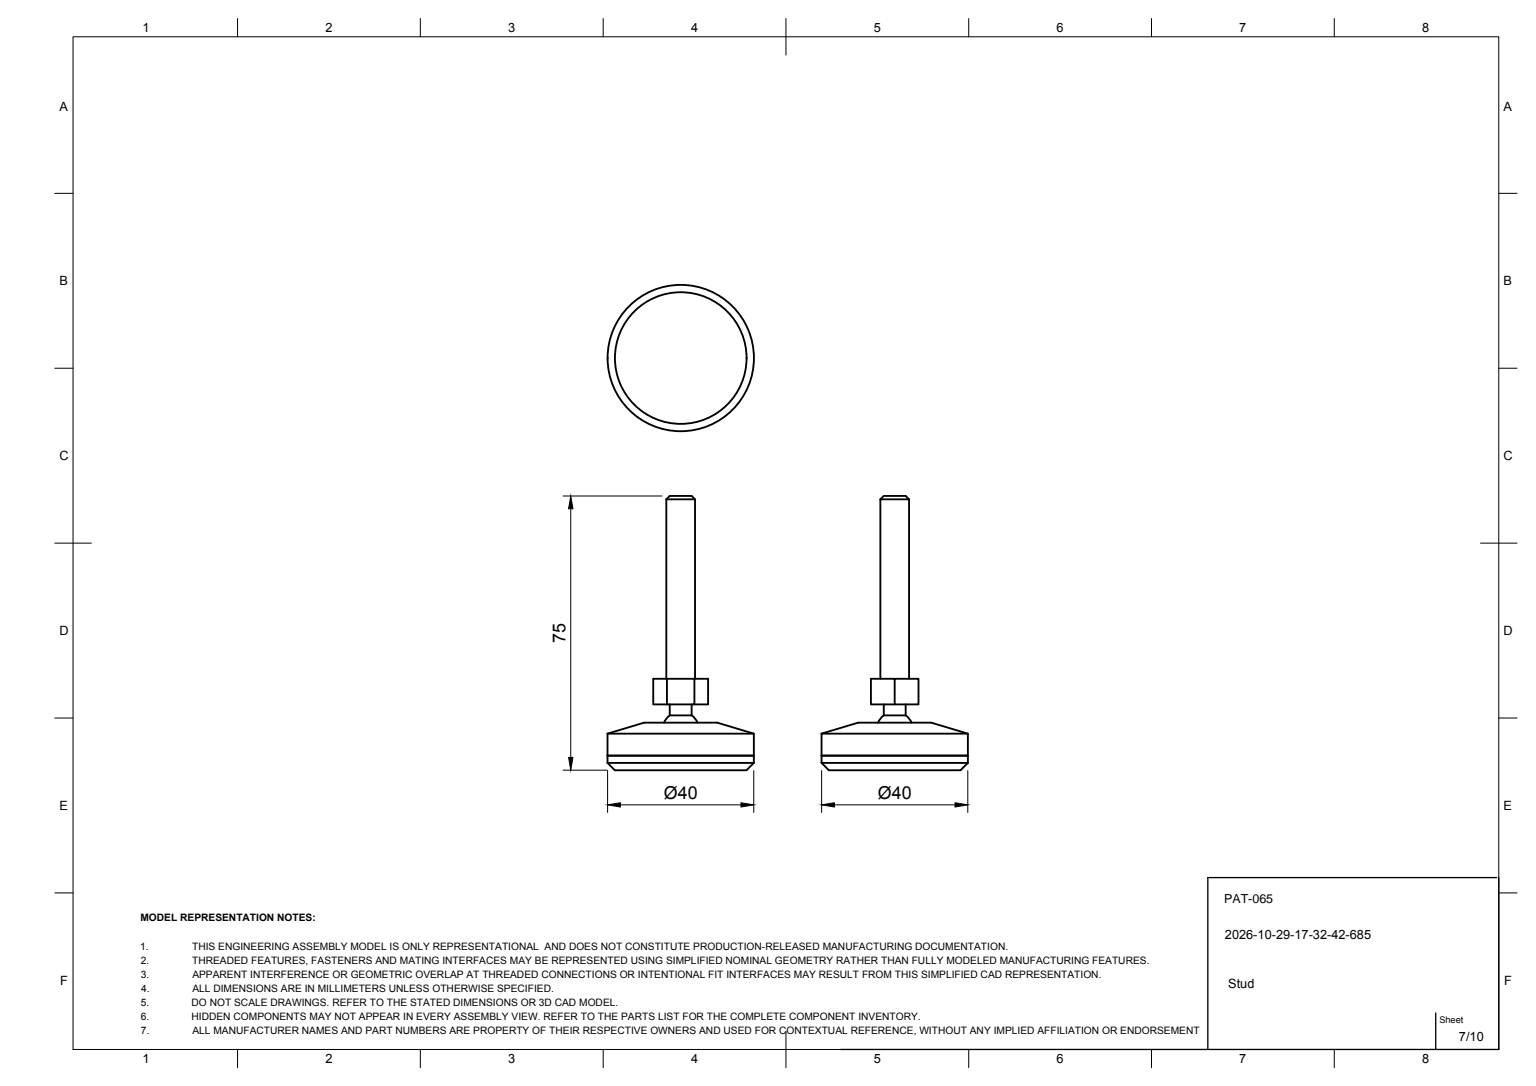
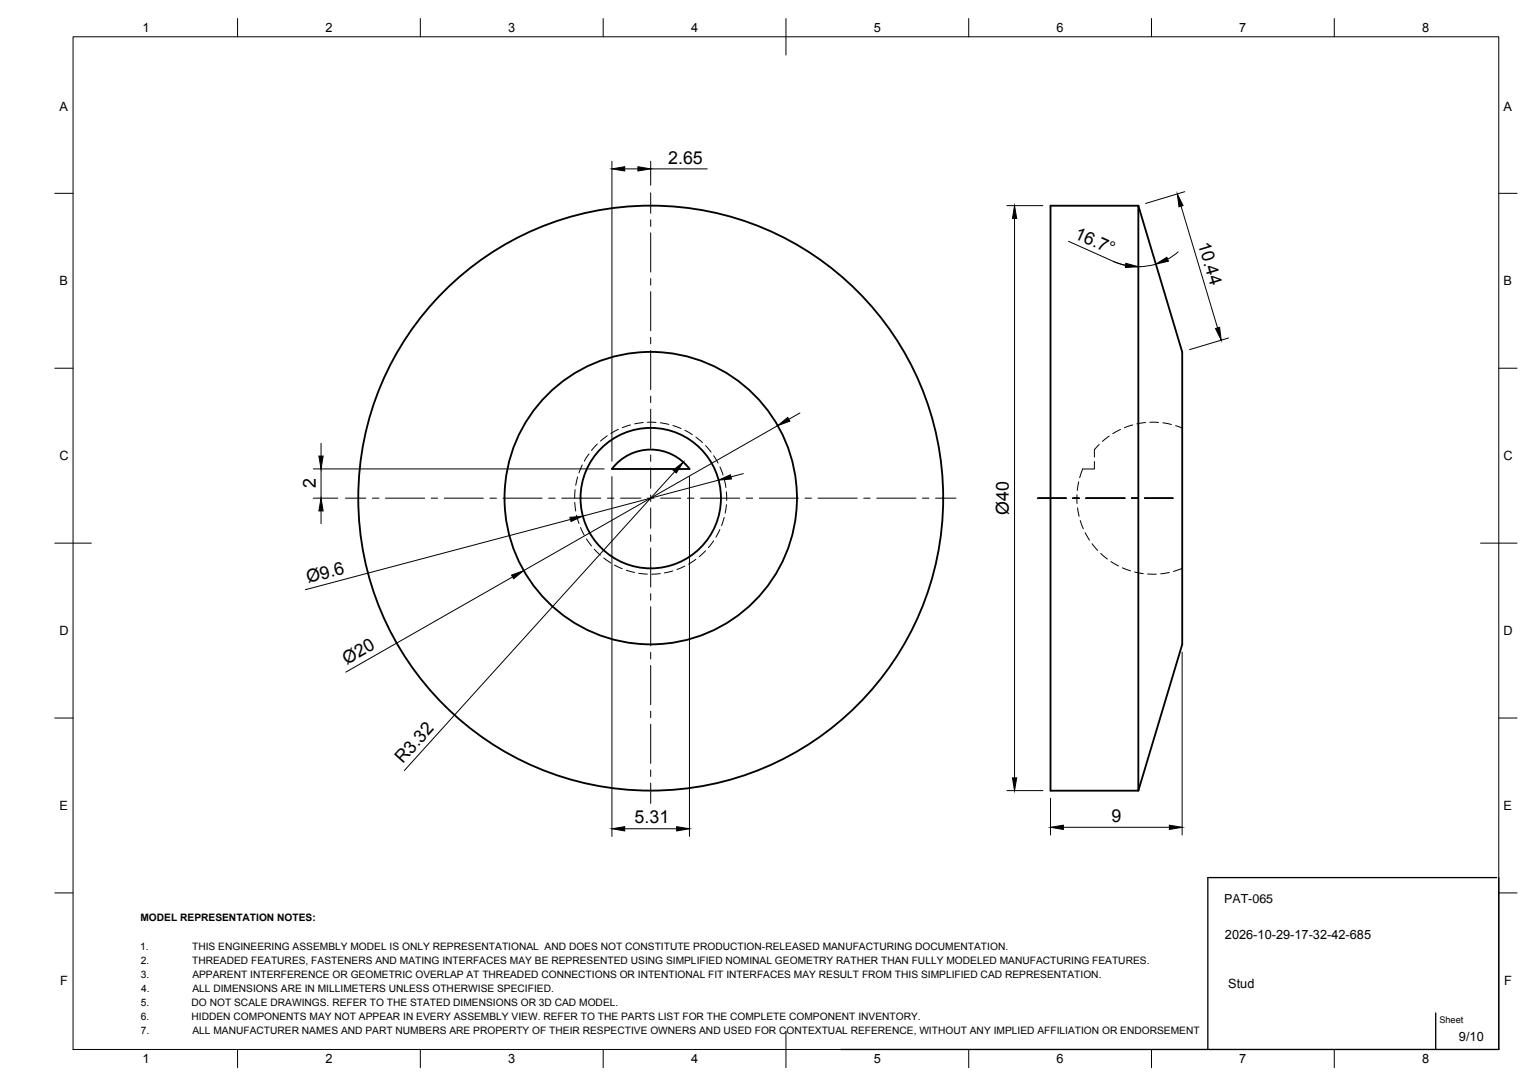
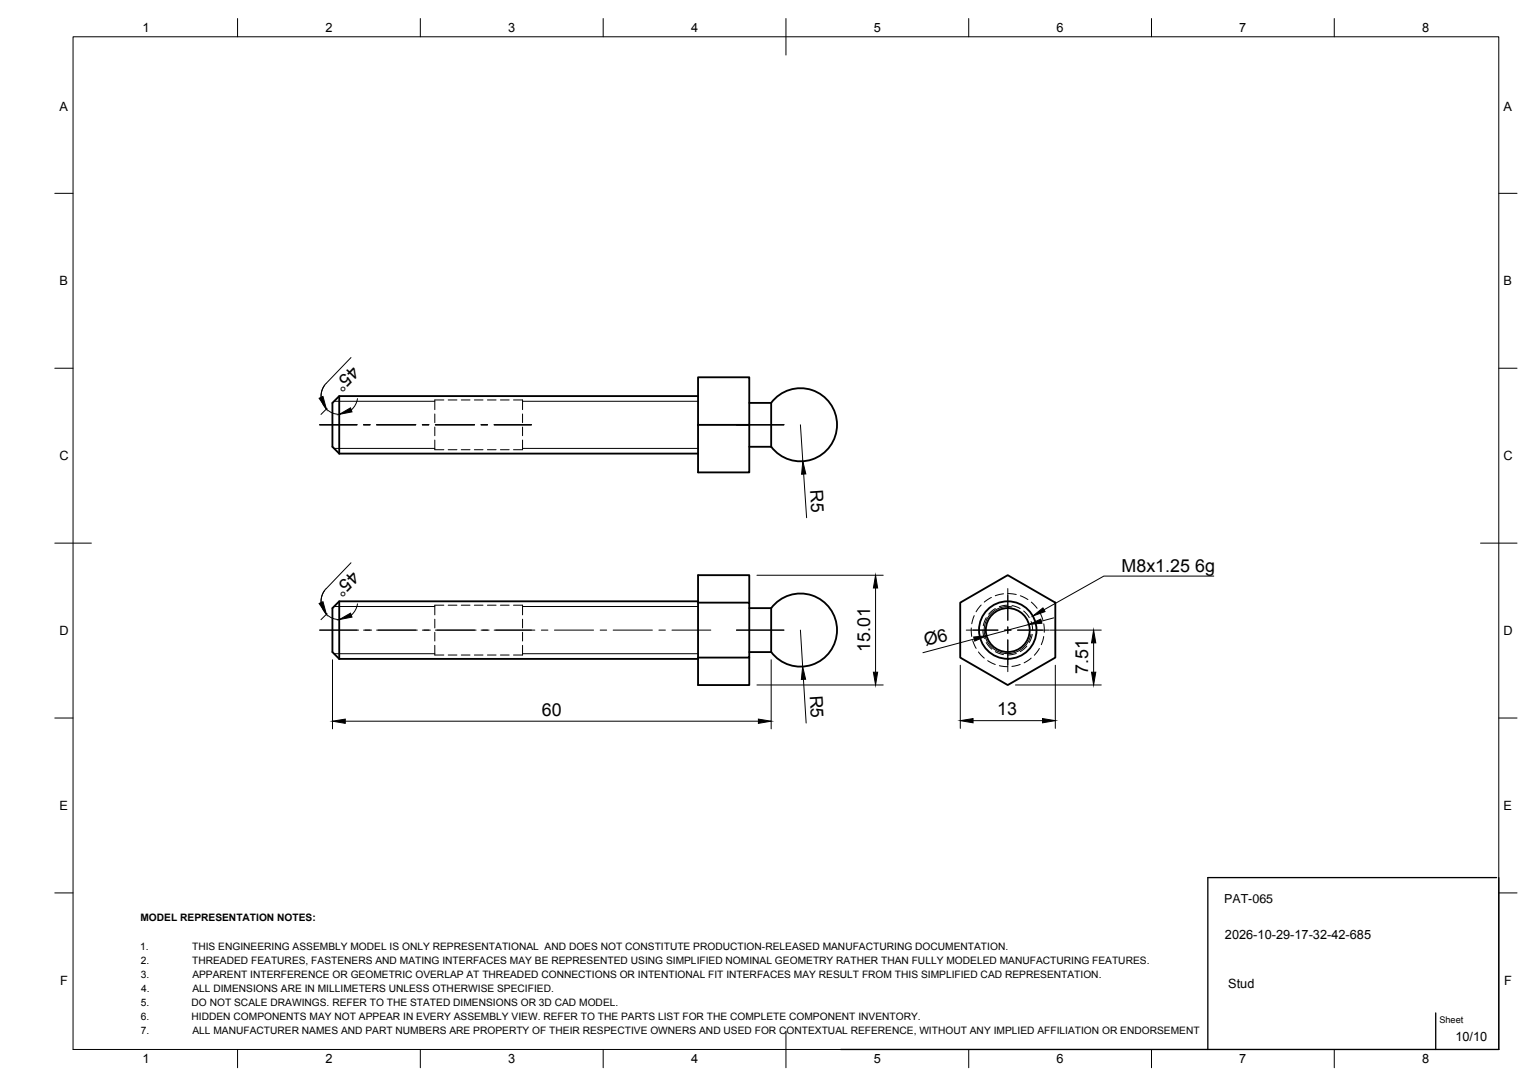
ISO-10303-21;
HEADER;
/* Generated by software containing ST-Developer
 * from STEP Tools, Inc. (www.steptools.com) 
 */

FILE_DESCRIPTION(
/* description */ ('PAT-065'),
/* implementation_level */ '2;1');

FILE_NAME(
/* name */ 'Stud.step',
/* time_stamp */ '2026-10-28T22:09:22-07:00',
/* author */ (''),
/* organization */ (''),
/* preprocessor_version */ 'ST-DEVELOPER v20.2',
/* originating_system */ 'Autodesk Translation Framework v15.17.0.0',
/* authorisation */ '');

FILE_SCHEMA (('AUTOMOTIVE_DESIGN { 1 0 10303 214 3 1 1 }'));
ENDSEC;

DATA;
#10=MECHANICAL_DESIGN_GEOMETRIC_PRESENTATION_REPRESENTATION('',(#164),#5502);
#115=ORIENTED_CLOSED_SHELL('',*,#3212,.F.);
#116=BREP_WITH_VOIDS('Body1',#3211,(#115));
#118=SPHERICAL_SURFACE('',#3514,0.5);
#123=CONICAL_SURFACE('',#3511,0.35,0.78539816339745);
#144=SHAPE_REPRESENTATION_RELATIONSHIP('SRR','None',#5562,#154);
#154=ADVANCED_BREP_SHAPE_REPRESENTATION('',(#116),#5498);
#164=STYLED_ITEM('',(#5701),#116);
#193=FACE_BOUND('',#641,.T.);
#194=FACE_BOUND('',#650,.T.);
#293=PLANE('',#3497);
#294=PLANE('',#3499);
#295=PLANE('',#3500);
#296=PLANE('',#3501);
#297=PLANE('',#3502);
#298=PLANE('',#3503);
#299=PLANE('',#3504);
#300=PLANE('',#3508);
#301=PLANE('',#3513);
#302=PLANE('',#3519);
#303=PLANE('',#3520);
#450=FACE_OUTER_BOUND('',#640,.T.);
#451=FACE_OUTER_BOUND('',#642,.T.);
#452=FACE_OUTER_BOUND('',#643,.T.);
#453=FACE_OUTER_BOUND('',#644,.T.);
#454=FACE_OUTER_BOUND('',#645,.T.);
#455=FACE_OUTER_BOUND('',#646,.T.);
#456=FACE_OUTER_BOUND('',#647,.T.);
#457=FACE_OUTER_BOUND('',#648,.T.);
#458=FACE_OUTER_BOUND('',#649,.T.);
#459=FACE_OUTER_BOUND('',#651,.T.);
#460=FACE_OUTER_BOUND('',#652,.T.);
#461=FACE_OUTER_BOUND('',#653,.T.);
#462=FACE_OUTER_BOUND('',#654,.T.);
#463=FACE_OUTER_BOUND('',#655,.T.);
#464=FACE_OUTER_BOUND('',#656,.T.);
#465=FACE_OUTER_BOUND('',#657,.T.);
#640=EDGE_LOOP('',(#2742,#2743,#2744,#2745,#2746,#2747));
#641=EDGE_LOOP('',(#2748));
#642=EDGE_LOOP('',(#2749,#2750,#2751,#2752));
#643=EDGE_LOOP('',(#2753,#2754,#2755,#2756));
#644=EDGE_LOOP('',(#2757,#2758,#2759,#2760));
#645=EDGE_LOOP('',(#2761,#2762,#2763,#2764));
#646=EDGE_LOOP('',(#2765,#2766,#2767,#2768));
#647=EDGE_LOOP('',(#2769,#2770,#2771,#2772));
#648=EDGE_LOOP('',(#2773,#2774,#2775,#2776));
#649=EDGE_LOOP('',(#2777,#2778,#2779,#2780,#2781,#2782));
#650=EDGE_LOOP('',(#2783));
#651=EDGE_LOOP('',(#2784,#2785,#2786,#2787));
#652=EDGE_LOOP('',(#2788,#2789,#2790,#2791));
#653=EDGE_LOOP('',(#2792));
#654=EDGE_LOOP('',(#2793,#2794,#2795));
#655=EDGE_LOOP('',(#2796,#2797,#2798,#2799));
#656=EDGE_LOOP('',(#2800));
#657=EDGE_LOOP('',(#2801));
#955=LINE('',#5152,#1286);
#956=LINE('',#5154,#1287);
#957=LINE('',#5156,#1288);
#958=LINE('',#5158,#1289);
#959=LINE('',#5160,#1290);
#960=LINE('',#5161,#1291);
#961=LINE('',#5167,#1292);
#962=LINE('',#5168,#1293);
#963=LINE('',#5169,#1294);
#964=LINE('',#5172,#1295);
#965=LINE('',#5173,#1296);
#966=LINE('',#5176,#1297);
#967=LINE('',#5177,#1298);
#968=LINE('',#5180,#1299);
#969=LINE('',#5181,#1300);
#970=LINE('',#5184,#1301);
#971=LINE('',#5185,#1302);
#972=LINE('',#5187,#1303);
#973=LINE('',#5192,#1304);
#974=LINE('',#5198,#1305);
#975=LINE('',#5202,#1306);
#976=LINE('',#5211,#1307);
#1286=VECTOR('',#4206,1.);
#1287=VECTOR('',#4207,1.);
#1288=VECTOR('',#4208,1.);
#1289=VECTOR('',#4209,1.);
#1290=VECTOR('',#4210,1.);
#1291=VECTOR('',#4211,1.);
#1292=VECTOR('',#4216,1.);
#1293=VECTOR('',#4217,1.);
#1294=VECTOR('',#4218,1.);
#1295=VECTOR('',#4221,1.);
#1296=VECTOR('',#4222,1.);
#1297=VECTOR('',#4225,1.);
#1298=VECTOR('',#4226,1.);
#1299=VECTOR('',#4229,1.);
#1300=VECTOR('',#4230,1.);
#1301=VECTOR('',#4233,1.);
#1302=VECTOR('',#4234,1.);
#1303=VECTOR('',#4237,1.);
#1304=VECTOR('',#4242,0.3);
#1305=VECTOR('',#4251,0.4);
#1306=VECTOR('',#4256,0.35);
#1307=VECTOR('',#4267,0.34);
#1415=CIRCLE('',#3498,0.3933);
#1416=CIRCLE('',#3506,0.3);
#1417=CIRCLE('',#3507,0.3);
#1418=CIRCLE('',#3510,0.3933);
#1419=CIRCLE('',#3512,0.3);
#1420=CIRCLE('',#3515,0.5);
#1421=CIRCLE('',#3517,0.34);
#1422=CIRCLE('',#3518,0.34);
#1640=VERTEX_POINT('',#5150);
#1641=VERTEX_POINT('',#5151);
#1642=VERTEX_POINT('',#5153);
#1643=VERTEX_POINT('',#5155);
#1644=VERTEX_POINT('',#5157);
#1645=VERTEX_POINT('',#5159);
#1646=VERTEX_POINT('',#5162);
#1647=VERTEX_POINT('',#5165);
#1648=VERTEX_POINT('',#5166);
#1649=VERTEX_POINT('',#5171);
#1650=VERTEX_POINT('',#5175);
#1651=VERTEX_POINT('',#5179);
#1652=VERTEX_POINT('',#5183);
#1653=VERTEX_POINT('',#5189);
#1654=VERTEX_POINT('',#5191);
#1655=VERTEX_POINT('',#5196);
#1656=VERTEX_POINT('',#5200);
#1657=VERTEX_POINT('',#5205);
#1658=VERTEX_POINT('',#5208);
#1659=VERTEX_POINT('',#5210);
#2021=EDGE_CURVE('',#1640,#1641,#955,.T.);
#2022=EDGE_CURVE('',#1641,#1642,#956,.T.);
#2023=EDGE_CURVE('',#1642,#1643,#957,.T.);
#2024=EDGE_CURVE('',#1643,#1644,#958,.T.);
#2025=EDGE_CURVE('',#1644,#1645,#959,.T.);
#2026=EDGE_CURVE('',#1645,#1640,#960,.T.);
#2027=EDGE_CURVE('',#1646,#1646,#1415,.F.);
#2028=EDGE_CURVE('',#1647,#1648,#961,.T.);
#2029=EDGE_CURVE('',#1648,#1640,#962,.T.);
#2030=EDGE_CURVE('',#1647,#1645,#963,.T.);
#2031=EDGE_CURVE('',#1649,#1647,#964,.T.);
#2032=EDGE_CURVE('',#1649,#1644,#965,.T.);
#2033=EDGE_CURVE('',#1650,#1649,#966,.T.);
#2034=EDGE_CURVE('',#1650,#1643,#967,.T.);
#2035=EDGE_CURVE('',#1651,#1650,#968,.T.);
#2036=EDGE_CURVE('',#1651,#1642,#969,.T.);
#2037=EDGE_CURVE('',#1652,#1651,#970,.T.);
#2038=EDGE_CURVE('',#1652,#1641,#971,.T.);
#2039=EDGE_CURVE('',#1648,#1652,#972,.T.);
#2040=EDGE_CURVE('',#1653,#1653,#1416,.T.);
#2041=EDGE_CURVE('',#1653,#1654,#973,.T.);
#2042=EDGE_CURVE('',#1654,#1654,#1417,.T.);
#2043=EDGE_CURVE('',#1655,#1655,#1418,.F.);
#2044=EDGE_CURVE('',#1655,#1646,#974,.T.);
#2045=EDGE_CURVE('',#1656,#1656,#1419,.T.);
#2046=EDGE_CURVE('',#1656,#1655,#975,.T.);
#2047=EDGE_CURVE('',#1654,#1657,#1420,.T.);
#2048=EDGE_CURVE('',#1658,#1658,#1421,.T.);
#2049=EDGE_CURVE('',#1658,#1659,#976,.T.);
#2050=EDGE_CURVE('',#1659,#1659,#1422,.T.);
#2742=ORIENTED_EDGE('',*,*,#2021,.T.);
#2743=ORIENTED_EDGE('',*,*,#2022,.T.);
#2744=ORIENTED_EDGE('',*,*,#2023,.T.);
#2745=ORIENTED_EDGE('',*,*,#2024,.T.);
#2746=ORIENTED_EDGE('',*,*,#2025,.T.);
#2747=ORIENTED_EDGE('',*,*,#2026,.T.);
#2748=ORIENTED_EDGE('',*,*,#2027,.F.);
#2749=ORIENTED_EDGE('',*,*,#2028,.T.);
#2750=ORIENTED_EDGE('',*,*,#2029,.T.);
#2751=ORIENTED_EDGE('',*,*,#2026,.F.);
#2752=ORIENTED_EDGE('',*,*,#2030,.F.);
#2753=ORIENTED_EDGE('',*,*,#2031,.T.);
#2754=ORIENTED_EDGE('',*,*,#2030,.T.);
#2755=ORIENTED_EDGE('',*,*,#2025,.F.);
#2756=ORIENTED_EDGE('',*,*,#2032,.F.);
#2757=ORIENTED_EDGE('',*,*,#2033,.T.);
#2758=ORIENTED_EDGE('',*,*,#2032,.T.);
#2759=ORIENTED_EDGE('',*,*,#2024,.F.);
#2760=ORIENTED_EDGE('',*,*,#2034,.F.);
#2761=ORIENTED_EDGE('',*,*,#2035,.T.);
#2762=ORIENTED_EDGE('',*,*,#2034,.T.);
#2763=ORIENTED_EDGE('',*,*,#2023,.F.);
#2764=ORIENTED_EDGE('',*,*,#2036,.F.);
#2765=ORIENTED_EDGE('',*,*,#2037,.T.);
#2766=ORIENTED_EDGE('',*,*,#2036,.T.);
#2767=ORIENTED_EDGE('',*,*,#2022,.F.);
#2768=ORIENTED_EDGE('',*,*,#2038,.F.);
#2769=ORIENTED_EDGE('',*,*,#2039,.T.);
#2770=ORIENTED_EDGE('',*,*,#2038,.T.);
#2771=ORIENTED_EDGE('',*,*,#2021,.F.);
#2772=ORIENTED_EDGE('',*,*,#2029,.F.);
#2773=ORIENTED_EDGE('',*,*,#2040,.F.);
#2774=ORIENTED_EDGE('',*,*,#2041,.T.);
#2775=ORIENTED_EDGE('',*,*,#2042,.F.);
#2776=ORIENTED_EDGE('',*,*,#2041,.F.);
#2777=ORIENTED_EDGE('',*,*,#2039,.F.);
#2778=ORIENTED_EDGE('',*,*,#2028,.F.);
#2779=ORIENTED_EDGE('',*,*,#2031,.F.);
#2780=ORIENTED_EDGE('',*,*,#2033,.F.);
#2781=ORIENTED_EDGE('',*,*,#2035,.F.);
#2782=ORIENTED_EDGE('',*,*,#2037,.F.);
#2783=ORIENTED_EDGE('',*,*,#2040,.T.);
#2784=ORIENTED_EDGE('',*,*,#2043,.F.);
#2785=ORIENTED_EDGE('',*,*,#2044,.T.);
#2786=ORIENTED_EDGE('',*,*,#2027,.T.);
#2787=ORIENTED_EDGE('',*,*,#2044,.F.);
#2788=ORIENTED_EDGE('',*,*,#2045,.F.);
#2789=ORIENTED_EDGE('',*,*,#2046,.T.);
#2790=ORIENTED_EDGE('',*,*,#2043,.T.);
#2791=ORIENTED_EDGE('',*,*,#2046,.F.);
#2792=ORIENTED_EDGE('',*,*,#2045,.T.);
#2793=ORIENTED_EDGE('',*,*,#2042,.T.);
#2794=ORIENTED_EDGE('',*,*,#2047,.T.);
#2795=ORIENTED_EDGE('',*,*,#2047,.F.);
#2796=ORIENTED_EDGE('',*,*,#2048,.F.);
#2797=ORIENTED_EDGE('',*,*,#2049,.T.);
#2798=ORIENTED_EDGE('',*,*,#2050,.T.);
#2799=ORIENTED_EDGE('',*,*,#2049,.F.);
#2800=ORIENTED_EDGE('',*,*,#2050,.F.);
#2801=ORIENTED_EDGE('',*,*,#2048,.T.);
#3020=CYLINDRICAL_SURFACE('',#3505,0.3);
#3021=CYLINDRICAL_SURFACE('',#3509,0.3933);
#3022=CYLINDRICAL_SURFACE('',#3516,0.34);
#3144=ADVANCED_FACE('',(#450,#193),#293,.T.);
#3145=ADVANCED_FACE('',(#451),#294,.T.);
#3146=ADVANCED_FACE('',(#452),#295,.T.);
#3147=ADVANCED_FACE('',(#453),#296,.T.);
#3148=ADVANCED_FACE('',(#454),#297,.T.);
#3149=ADVANCED_FACE('',(#455),#298,.T.);
#3150=ADVANCED_FACE('',(#456),#299,.T.);
#3151=ADVANCED_FACE('',(#457),#3020,.T.);
#3152=ADVANCED_FACE('',(#458,#194),#300,.T.);
#3153=ADVANCED_FACE('',(#459),#3021,.T.);
#3154=ADVANCED_FACE('',(#460),#123,.T.);
#3155=ADVANCED_FACE('',(#461),#301,.T.);
#3156=ADVANCED_FACE('',(#462),#118,.T.);
#3157=ADVANCED_FACE('',(#463),#3022,.F.);
#3158=ADVANCED_FACE('',(#464),#302,.F.);
#3159=ADVANCED_FACE('',(#465),#303,.T.);
#3211=CLOSED_SHELL('',(#3144,#3145,#3146,#3147,#3148,#3149,#3150,#3151,
#3152,#3153,#3154,#3155,#3156));
#3212=CLOSED_SHELL('',(#3157,#3158,#3159));
#3496=AXIS2_PLACEMENT_3D('',#5148,#4202,#4203);
#3497=AXIS2_PLACEMENT_3D('',#5149,#4204,#4205);
#3498=AXIS2_PLACEMENT_3D('',#5163,#4212,#4213);
#3499=AXIS2_PLACEMENT_3D('',#5164,#4214,#4215);
#3500=AXIS2_PLACEMENT_3D('',#5170,#4219,#4220);
#3501=AXIS2_PLACEMENT_3D('',#5174,#4223,#4224);
#3502=AXIS2_PLACEMENT_3D('',#5178,#4227,#4228);
#3503=AXIS2_PLACEMENT_3D('',#5182,#4231,#4232);
#3504=AXIS2_PLACEMENT_3D('',#5186,#4235,#4236);
#3505=AXIS2_PLACEMENT_3D('',#5188,#4238,#4239);
#3506=AXIS2_PLACEMENT_3D('',#5190,#4240,#4241);
#3507=AXIS2_PLACEMENT_3D('',#5193,#4243,#4244);
#3508=AXIS2_PLACEMENT_3D('',#5194,#4245,#4246);
#3509=AXIS2_PLACEMENT_3D('',#5195,#4247,#4248);
#3510=AXIS2_PLACEMENT_3D('',#5197,#4249,#4250);
#3511=AXIS2_PLACEMENT_3D('',#5199,#4252,#4253);
#3512=AXIS2_PLACEMENT_3D('',#5201,#4254,#4255);
#3513=AXIS2_PLACEMENT_3D('',#5203,#4257,#4258);
#3514=AXIS2_PLACEMENT_3D('',#5204,#4259,#4260);
#3515=AXIS2_PLACEMENT_3D('',#5206,#4261,#4262);
#3516=AXIS2_PLACEMENT_3D('',#5207,#4263,#4264);
#3517=AXIS2_PLACEMENT_3D('',#5209,#4265,#4266);
#3518=AXIS2_PLACEMENT_3D('',#5212,#4268,#4269);
#3519=AXIS2_PLACEMENT_3D('',#5213,#4270,#4271);
#3520=AXIS2_PLACEMENT_3D('',#5214,#4272,#4273);
#4202=DIRECTION('axis',(0.,0.,1.));
#4203=DIRECTION('refdir',(1.,0.,0.));
#4204=DIRECTION('center_axis',(0.,0.,1.));
#4205=DIRECTION('ref_axis',(1.,0.,0.));
#4206=DIRECTION('',(0.5,0.866025403784439,0.));
#4207=DIRECTION('',(-0.5,0.866025403784439,0.));
#4208=DIRECTION('',(-1.,1.4792020664489E-16,0.));
#4209=DIRECTION('',(-0.5,-0.866025403784439,0.));
#4210=DIRECTION('',(0.5,-0.866025403784439,0.));
#4211=DIRECTION('',(1.,-2.95840413289779E-16,0.));
#4212=DIRECTION('center_axis',(0.,0.,-1.));
#4213=DIRECTION('ref_axis',(1.,0.,0.));
#4214=DIRECTION('center_axis',(-2.95840413289779E-16,-1.,0.));
#4215=DIRECTION('ref_axis',(1.,-2.95840413289779E-16,0.));
#4216=DIRECTION('',(1.,-2.95840413289779E-16,0.));
#4217=DIRECTION('',(0.,0.,1.));
#4218=DIRECTION('',(0.,0.,1.));
#4219=DIRECTION('center_axis',(-0.866025403784439,-0.5,0.));
#4220=DIRECTION('ref_axis',(0.5,-0.866025403784439,0.));
#4221=DIRECTION('',(0.5,-0.866025403784439,0.));
#4222=DIRECTION('',(0.,0.,1.));
#4223=DIRECTION('center_axis',(-0.866025403784439,0.5,0.));
#4224=DIRECTION('ref_axis',(-0.5,-0.866025403784439,0.));
#4225=DIRECTION('',(-0.5,-0.866025403784439,0.));
#4226=DIRECTION('',(0.,0.,1.));
#4227=DIRECTION('center_axis',(1.4792020664489E-16,1.,0.));
#4228=DIRECTION('ref_axis',(-1.,1.4792020664489E-16,0.));
#4229=DIRECTION('',(-1.,1.4792020664489E-16,0.));
#4230=DIRECTION('',(0.,0.,1.));
#4231=DIRECTION('center_axis',(0.866025403784439,0.5,0.));
#4232=DIRECTION('ref_axis',(-0.5,0.866025403784439,0.));
#4233=DIRECTION('',(-0.5,0.866025403784439,0.));
#4234=DIRECTION('',(0.,0.,1.));
#4235=DIRECTION('center_axis',(0.866025403784439,-0.5,0.));
#4236=DIRECTION('ref_axis',(0.5,0.866025403784439,0.));
#4237=DIRECTION('',(0.5,0.866025403784439,0.));
#4238=DIRECTION('center_axis',(0.,0.,1.));
#4239=DIRECTION('ref_axis',(1.,0.,0.));
#4240=DIRECTION('center_axis',(0.,0.,1.));
#4241=DIRECTION('ref_axis',(1.,0.,0.));
#4242=DIRECTION('',(0.,0.,-1.));
#4243=DIRECTION('center_axis',(0.,0.,-1.));
#4244=DIRECTION('ref_axis',(1.,0.,0.));
#4245=DIRECTION('center_axis',(0.,0.,-1.));
#4246=DIRECTION('ref_axis',(-1.,0.,0.));
#4247=DIRECTION('center_axis',(0.,0.,1.));
#4248=DIRECTION('ref_axis',(1.,0.,0.));
#4249=DIRECTION('center_axis',(0.,0.,-1.));
#4250=DIRECTION('ref_axis',(1.,0.,0.));
#4251=DIRECTION('',(0.,0.,-1.));
#4252=DIRECTION('center_axis',(0.,0.,-1.));
#4253=DIRECTION('ref_axis',(1.,0.,0.));
#4254=DIRECTION('center_axis',(0.,0.,1.));
#4255=DIRECTION('ref_axis',(1.,0.,0.));
#4256=DIRECTION('',(-0.707106781186549,-8.65956056235495E-17,-0.707106781186546));
#4257=DIRECTION('center_axis',(0.,0.,1.));
#4258=DIRECTION('ref_axis',(1.,0.,0.));
#4259=DIRECTION('center_axis',(6.12323399573677E-17,0.,1.));
#4260=DIRECTION('ref_axis',(1.,0.,0.));
#4261=DIRECTION('center_axis',(1.22464679914735E-16,-1.,0.));
#4262=DIRECTION('ref_axis',(-1.,-1.22464679914735E-16,0.));
#4263=DIRECTION('center_axis',(0.,0.,1.));
#4264=DIRECTION('ref_axis',(1.,0.,0.));
#4265=DIRECTION('center_axis',(0.,0.,1.));
#4266=DIRECTION('ref_axis',(1.,0.,0.));
#4267=DIRECTION('',(0.,0.,1.));
#4268=DIRECTION('center_axis',(0.,0.,1.));
#4269=DIRECTION('ref_axis',(1.,0.,0.));
#4270=DIRECTION('center_axis',(0.,0.,1.));
#4271=DIRECTION('ref_axis',(1.,0.,0.));
#4272=DIRECTION('center_axis',(0.,0.,1.));
#4273=DIRECTION('ref_axis',(1.,0.,0.));
#5148=CARTESIAN_POINT('',(0.,0.,0.));
#5149=CARTESIAN_POINT('Origin',(0.,1.11022302462516E-16,2.5));
#5150=CARTESIAN_POINT('',(0.375277674973257,-0.65,2.5));
#5151=CARTESIAN_POINT('',(0.750555349946514,0.,2.5));
#5152=CARTESIAN_POINT('',(0.375277674973257,-0.65,2.5));
#5153=CARTESIAN_POINT('',(0.375277674973257,0.65,2.5));
#5154=CARTESIAN_POINT('',(0.750555349946514,0.,2.5));
#5155=CARTESIAN_POINT('',(-0.375277674973257,0.65,2.5));
#5156=CARTESIAN_POINT('',(0.375277674973257,0.65,2.5));
#5157=CARTESIAN_POINT('',(-0.750555349946514,1.11022302462516E-16,2.5));
#5158=CARTESIAN_POINT('',(-0.375277674973257,0.65,2.5));
#5159=CARTESIAN_POINT('',(-0.375277674973257,-0.65,2.5));
#5160=CARTESIAN_POINT('',(-0.750555349946514,9.19165206894919E-17,2.5));
#5161=CARTESIAN_POINT('',(-0.375277674973257,-0.65,2.5));
#5162=CARTESIAN_POINT('',(-0.3933,4.81653586104654E-17,2.5));
#5163=CARTESIAN_POINT('Origin',(0.,0.,2.5));
#5164=CARTESIAN_POINT('Origin',(-0.375277674973257,-0.65,1.8));
#5165=CARTESIAN_POINT('',(-0.375277674973257,-0.65,1.8));
#5166=CARTESIAN_POINT('',(0.375277674973257,-0.65,1.8));
#5167=CARTESIAN_POINT('',(-0.375277674973257,-0.65,1.8));
#5168=CARTESIAN_POINT('',(0.375277674973257,-0.65,1.8));
#5169=CARTESIAN_POINT('',(-0.375277674973257,-0.65,1.8));
#5170=CARTESIAN_POINT('Origin',(-0.750555349946514,9.19165206894919E-17,
1.8));
#5171=CARTESIAN_POINT('',(-0.750555349946514,9.19165206894919E-17,1.8));
#5172=CARTESIAN_POINT('',(-0.750555349946514,9.19165206894919E-17,1.8));
#5173=CARTESIAN_POINT('',(-0.750555349946514,9.19165206894919E-17,1.8));
#5174=CARTESIAN_POINT('Origin',(-0.375277674973257,0.65,1.8));
#5175=CARTESIAN_POINT('',(-0.375277674973257,0.65,1.8));
#5176=CARTESIAN_POINT('',(-0.375277674973257,0.65,1.8));
#5177=CARTESIAN_POINT('',(-0.375277674973257,0.65,1.8));
#5178=CARTESIAN_POINT('Origin',(0.375277674973257,0.65,1.8));
#5179=CARTESIAN_POINT('',(0.375277674973257,0.65,1.8));
#5180=CARTESIAN_POINT('',(0.375277674973257,0.65,1.8));
#5181=CARTESIAN_POINT('',(0.375277674973257,0.65,1.8));
#5182=CARTESIAN_POINT('Origin',(0.750555349946514,0.,1.8));
#5183=CARTESIAN_POINT('',(0.750555349946514,0.,1.8));
#5184=CARTESIAN_POINT('',(0.750555349946514,0.,1.8));
#5185=CARTESIAN_POINT('',(0.750555349946514,0.,1.8));
#5186=CARTESIAN_POINT('Origin',(0.375277674973257,-0.65,1.8));
#5187=CARTESIAN_POINT('',(0.375277674973257,-0.65,1.8));
#5188=CARTESIAN_POINT('Origin',(0.,0.,1.45));
#5189=CARTESIAN_POINT('',(-0.3,-3.67394039744206E-17,1.8));
#5190=CARTESIAN_POINT('Origin',(0.,0.,1.8));
#5191=CARTESIAN_POINT('',(-0.3,3.67394039744206E-17,1.5));
#5192=CARTESIAN_POINT('',(-0.3,-3.67394039744206E-17,1.45));
#5193=CARTESIAN_POINT('Origin',(0.,0.,1.5));
#5194=CARTESIAN_POINT('Origin',(0.4,0.,1.8));
#5195=CARTESIAN_POINT('Origin',(0.,0.,4.6));
#5196=CARTESIAN_POINT('',(-0.3933,4.81653586104654E-17,7.4067));
#5197=CARTESIAN_POINT('Origin',(0.,0.,7.4067));
#5198=CARTESIAN_POINT('',(-0.3933,-4.81653586104654E-17,4.6));
#5199=CARTESIAN_POINT('Origin',(0.,0.,7.45));
#5200=CARTESIAN_POINT('',(-0.3,-3.67394039744206E-17,7.5));
#5201=CARTESIAN_POINT('Origin',(0.,0.,7.5));
#5202=CARTESIAN_POINT('',(-0.35,-4.28626379701574E-17,7.45));
#5203=CARTESIAN_POINT('Origin',(0.,0.,7.5));
#5204=CARTESIAN_POINT('Origin',(-5.55111512312578E-17,0.,1.1));
#5205=CARTESIAN_POINT('',(-8.61273212099417E-17,-3.74939945665464E-33,0.6));
#5206=CARTESIAN_POINT('Origin',(-5.55111512312578E-17,0.,1.1));
#5207=CARTESIAN_POINT('Origin',(0.,0.,4.9));
#5208=CARTESIAN_POINT('',(-0.34,-4.163799117101E-17,4.9));
#5209=CARTESIAN_POINT('Origin',(0.,0.,4.9));
#5210=CARTESIAN_POINT('',(-0.34,-4.163799117101E-17,6.1));
#5211=CARTESIAN_POINT('',(-0.34,-4.163799117101E-17,4.9));
#5212=CARTESIAN_POINT('Origin',(0.,0.,6.1));
#5213=CARTESIAN_POINT('Origin',(0.,0.,6.1));
#5214=CARTESIAN_POINT('Origin',(0.,0.,4.9));
#5485=UNCERTAINTY_MEASURE_WITH_UNIT(LENGTH_MEASURE(0.001),#5503,
'DISTANCE_ACCURACY_VALUE',
'Maximum model space distance between geometric entities at asserted c
onnectivities');
#5489=UNCERTAINTY_MEASURE_WITH_UNIT(LENGTH_MEASURE(0.001),#5503,
'DISTANCE_ACCURACY_VALUE',
'Maximum model space distance between geometric entities at asserted c
onnectivities');
#5498=(
GEOMETRIC_REPRESENTATION_CONTEXT(3)
GLOBAL_UNCERTAINTY_ASSIGNED_CONTEXT((#5485))
GLOBAL_UNIT_ASSIGNED_CONTEXT((#5503,#5505,#5506))
REPRESENTATION_CONTEXT('','3D')
);
#5502=(
GEOMETRIC_REPRESENTATION_CONTEXT(3)
GLOBAL_UNCERTAINTY_ASSIGNED_CONTEXT((#5489))
GLOBAL_UNIT_ASSIGNED_CONTEXT((#5503,#5505,#5506))
REPRESENTATION_CONTEXT('','3D')
);
#5503=(
LENGTH_UNIT()
NAMED_UNIT(*)
SI_UNIT(.CENTI.,.METRE.)
);
#5505=(
NAMED_UNIT(*)
PLANE_ANGLE_UNIT()
SI_UNIT($,.RADIAN.)
);
#5506=(
NAMED_UNIT(*)
SI_UNIT($,.STERADIAN.)
SOLID_ANGLE_UNIT()
);
#5515=SHAPE_DEFINITION_REPRESENTATION(#5527,#5562);
#5527=PRODUCT_DEFINITION_SHAPE('',$,#5575);
#5562=SHAPE_REPRESENTATION('',(#3496),#5498);
#5566=PRODUCT_DEFINITION_CONTEXT('part definition',#5604,'design');
#5575=PRODUCT_DEFINITION('Stud','Stud',#5587,#5566);
#5587=PRODUCT_DEFINITION_FORMATION('',$,#5614);
#5604=APPLICATION_CONTEXT(
'Core Data for Automotive Mechanical Design Process');
#5605=PRODUCT_CONTEXT('part definition',#5604,'mechanical');
#5614=PRODUCT('Stud','Stud','Stud',(#5605));
#5695=COLOUR_RGB('Black',0.12,0.14,0.17);
#5696=FILL_AREA_STYLE_COLOUR('',#5695);
#5697=FILL_AREA_STYLE('',(#5696));
#5698=SURFACE_STYLE_FILL_AREA(#5697);
#5699=SURFACE_SIDE_STYLE('',(#5698));
#5700=SURFACE_STYLE_USAGE(.BOTH.,#5699);
#5701=PRESENTATION_STYLE_ASSIGNMENT((#5700));
ENDSEC;
END-ISO-10303-21;
